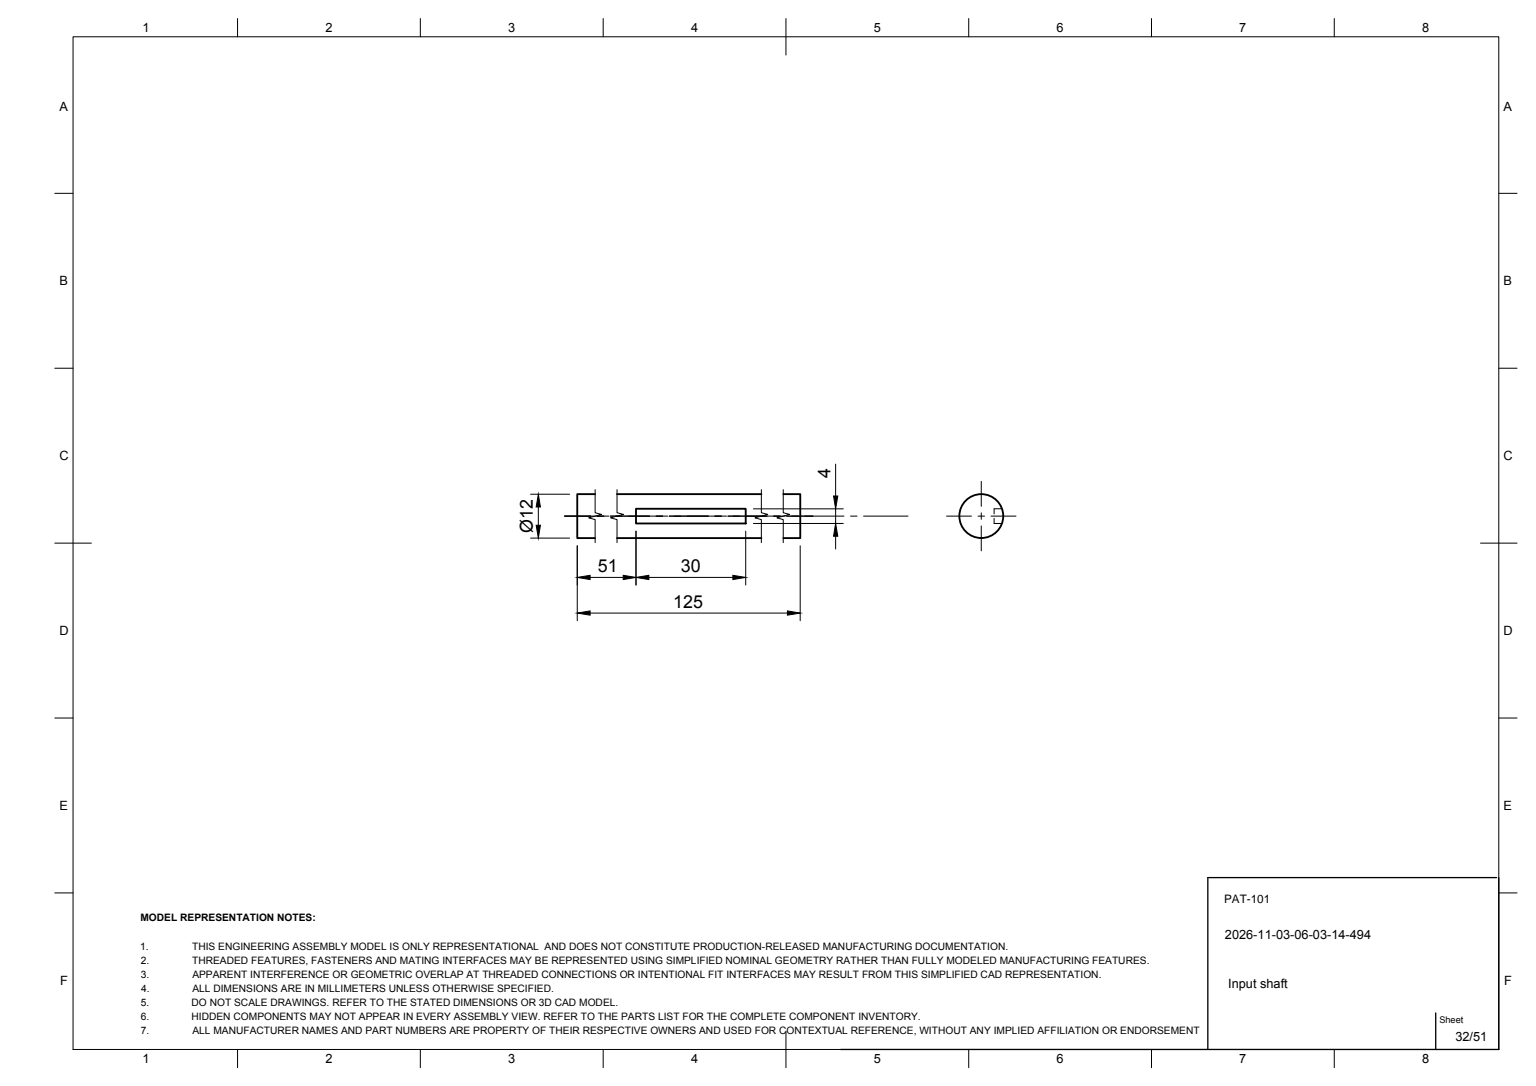
ISO-10303-21;
HEADER;
/* Generated by software containing ST-Developer
 * from STEP Tools, Inc. (www.steptools.com) 
 */

FILE_DESCRIPTION(
/* description */ ('Spur gear reduction stage 2-1 on bearing plates'),
/* implementation_level */ '2;1');

FILE_NAME(
/* name */ 'Input shaft.step',
/* time_stamp */ '2026-10-28T03:22:07-07:00',
/* author */ (''),
/* organization */ (''),
/* preprocessor_version */ 'ST-DEVELOPER v20.2',
/* originating_system */ 'Autodesk Translation Framework v15.17.0.0',
/* authorisation */ '');

FILE_SCHEMA (('AUTOMOTIVE_DESIGN { 1 0 10303 214 3 1 1 }'));
ENDSEC;

DATA;
#10=MECHANICAL_DESIGN_GEOMETRIC_PRESENTATION_REPRESENTATION('',(#986),#53909);
#885=SHAPE_REPRESENTATION_RELATIONSHIP('SRR','None',#54115,#928);
#928=ADVANCED_BREP_SHAPE_REPRESENTATION('',(#1041),#53889);
#986=STYLED_ITEM('',(#54397),#1041);
#1041=MANIFOLD_SOLID_BREP('Body1',#11313);
#1197=FACE_BOUND('',#2574,.T.);
#1358=PLANE('',#12482);
#1359=PLANE('',#12483);
#1360=PLANE('',#12485);
#1361=PLANE('',#12486);
#1362=PLANE('',#12487);
#1363=PLANE('',#12492);
#1364=PLANE('',#12493);
#1783=FACE_OUTER_BOUND('',#2568,.T.);
#1784=FACE_OUTER_BOUND('',#2569,.T.);
#1785=FACE_OUTER_BOUND('',#2570,.T.);
#1786=FACE_OUTER_BOUND('',#2571,.T.);
#1787=FACE_OUTER_BOUND('',#2572,.T.);
#1788=FACE_OUTER_BOUND('',#2573,.T.);
#1789=FACE_OUTER_BOUND('',#2575,.T.);
#1790=FACE_OUTER_BOUND('',#2576,.T.);
#2568=EDGE_LOOP('',(#8482,#8483,#8484,#8485));
#2569=EDGE_LOOP('',(#8486,#8487,#8488,#8489));
#2570=EDGE_LOOP('',(#8490,#8491,#8492,#8493));
#2571=EDGE_LOOP('',(#8494,#8495,#8496,#8497));
#2572=EDGE_LOOP('',(#8498,#8499,#8500,#8501));
#2573=EDGE_LOOP('',(#8502,#8503,#8504,#8505));
#2574=EDGE_LOOP('',(#8506,#8507,#8508,#8509));
#2575=EDGE_LOOP('',(#8510));
#2576=EDGE_LOOP('',(#8511));
#3193=LINE('',#17924,#3834);
#3194=LINE('',#17926,#3835);
#3195=LINE('',#17928,#3836);
#3196=LINE('',#17929,#3837);
#3197=LINE('',#17934,#3838);
#3198=LINE('',#17935,#3839);
#3199=LINE('',#17938,#3840);
#3200=LINE('',#17940,#3841);
#3201=LINE('',#17941,#3842);
#3202=LINE('',#17943,#3843);
#3203=LINE('',#17950,#3844);
#3834=VECTOR('',#14552,1.);
#3835=VECTOR('',#14553,1.);
#3836=VECTOR('',#14554,1.);
#3837=VECTOR('',#14555,1.);
#3838=VECTOR('',#14560,1.);
#3839=VECTOR('',#14561,1.);
#3840=VECTOR('',#14564,1.);
#3841=VECTOR('',#14565,1.);
#3842=VECTOR('',#14566,1.);
#3843=VECTOR('',#14569,1.);
#3844=VECTOR('',#14578,0.6);
#4576=CIRCLE('',#12484,0.6);
#4577=CIRCLE('',#12488,0.6);
#4578=CIRCLE('',#12490,0.6);
#4579=CIRCLE('',#12491,0.6);
#5174=VERTEX_POINT('',#17922);
#5175=VERTEX_POINT('',#17923);
#5176=VERTEX_POINT('',#17925);
#5177=VERTEX_POINT('',#17927);
#5178=VERTEX_POINT('',#17931);
#5179=VERTEX_POINT('',#17933);
#5180=VERTEX_POINT('',#17937);
#5181=VERTEX_POINT('',#17939);
#5182=VERTEX_POINT('',#17947);
#5183=VERTEX_POINT('',#17949);
#6383=EDGE_CURVE('',#5174,#5175,#3193,.T.);
#6384=EDGE_CURVE('',#5174,#5176,#3194,.T.);
#6385=EDGE_CURVE('',#5177,#5176,#3195,.T.);
#6386=EDGE_CURVE('',#5177,#5175,#3196,.T.);
#6387=EDGE_CURVE('',#5175,#5178,#4576,.T.);
#6388=EDGE_CURVE('',#5179,#5177,#3197,.T.);
#6389=EDGE_CURVE('',#5178,#5179,#3198,.T.);
#6390=EDGE_CURVE('',#5178,#5180,#3199,.T.);
#6391=EDGE_CURVE('',#5179,#5181,#3200,.T.);
#6392=EDGE_CURVE('',#5181,#5180,#3201,.T.);
#6393=EDGE_CURVE('',#5176,#5181,#3202,.T.);
#6394=EDGE_CURVE('',#5180,#5174,#4577,.T.);
#6395=EDGE_CURVE('',#5182,#5182,#4578,.T.);
#6396=EDGE_CURVE('',#5182,#5183,#3203,.T.);
#6397=EDGE_CURVE('',#5183,#5183,#4579,.T.);
#8482=ORIENTED_EDGE('',*,*,#6383,.F.);
#8483=ORIENTED_EDGE('',*,*,#6384,.T.);
#8484=ORIENTED_EDGE('',*,*,#6385,.F.);
#8485=ORIENTED_EDGE('',*,*,#6386,.T.);
#8486=ORIENTED_EDGE('',*,*,#6387,.F.);
#8487=ORIENTED_EDGE('',*,*,#6386,.F.);
#8488=ORIENTED_EDGE('',*,*,#6388,.F.);
#8489=ORIENTED_EDGE('',*,*,#6389,.F.);
#8490=ORIENTED_EDGE('',*,*,#6390,.F.);
#8491=ORIENTED_EDGE('',*,*,#6389,.T.);
#8492=ORIENTED_EDGE('',*,*,#6391,.T.);
#8493=ORIENTED_EDGE('',*,*,#6392,.T.);
#8494=ORIENTED_EDGE('',*,*,#6388,.T.);
#8495=ORIENTED_EDGE('',*,*,#6385,.T.);
#8496=ORIENTED_EDGE('',*,*,#6393,.T.);
#8497=ORIENTED_EDGE('',*,*,#6391,.F.);
#8498=ORIENTED_EDGE('',*,*,#6394,.F.);
#8499=ORIENTED_EDGE('',*,*,#6392,.F.);
#8500=ORIENTED_EDGE('',*,*,#6393,.F.);
#8501=ORIENTED_EDGE('',*,*,#6384,.F.);
#8502=ORIENTED_EDGE('',*,*,#6395,.F.);
#8503=ORIENTED_EDGE('',*,*,#6396,.T.);
#8504=ORIENTED_EDGE('',*,*,#6397,.T.);
#8505=ORIENTED_EDGE('',*,*,#6396,.F.);
#8506=ORIENTED_EDGE('',*,*,#6390,.T.);
#8507=ORIENTED_EDGE('',*,*,#6394,.T.);
#8508=ORIENTED_EDGE('',*,*,#6383,.T.);
#8509=ORIENTED_EDGE('',*,*,#6387,.T.);
#8510=ORIENTED_EDGE('',*,*,#6395,.T.);
#8511=ORIENTED_EDGE('',*,*,#6397,.F.);
#10526=CYLINDRICAL_SURFACE('',#12489,0.6);
#10903=ADVANCED_FACE('',(#1783),#1358,.F.);
#10904=ADVANCED_FACE('',(#1784),#1359,.T.);
#10905=ADVANCED_FACE('',(#1785),#1360,.F.);
#10906=ADVANCED_FACE('',(#1786),#1361,.F.);
#10907=ADVANCED_FACE('',(#1787),#1362,.F.);
#10908=ADVANCED_FACE('',(#1788,#1197),#10526,.T.);
#10909=ADVANCED_FACE('',(#1789),#1363,.T.);
#10910=ADVANCED_FACE('',(#1790),#1364,.F.);
#11313=CLOSED_SHELL('',(#10903,#10904,#10905,#10906,#10907,#10908,#10909,
#10910));
#12481=AXIS2_PLACEMENT_3D('',#17920,#14548,#14549);
#12482=AXIS2_PLACEMENT_3D('',#17921,#14550,#14551);
#12483=AXIS2_PLACEMENT_3D('',#17930,#14556,#14557);
#12484=AXIS2_PLACEMENT_3D('',#17932,#14558,#14559);
#12485=AXIS2_PLACEMENT_3D('',#17936,#14562,#14563);
#12486=AXIS2_PLACEMENT_3D('',#17942,#14567,#14568);
#12487=AXIS2_PLACEMENT_3D('',#17944,#14570,#14571);
#12488=AXIS2_PLACEMENT_3D('',#17945,#14572,#14573);
#12489=AXIS2_PLACEMENT_3D('',#17946,#14574,#14575);
#12490=AXIS2_PLACEMENT_3D('',#17948,#14576,#14577);
#12491=AXIS2_PLACEMENT_3D('',#17951,#14579,#14580);
#12492=AXIS2_PLACEMENT_3D('',#17952,#14581,#14582);
#12493=AXIS2_PLACEMENT_3D('',#17953,#14583,#14584);
#14548=DIRECTION('axis',(0.,0.,1.));
#14549=DIRECTION('refdir',(1.,0.,0.));
#14550=DIRECTION('center_axis',(-1.,0.,0.));
#14551=DIRECTION('ref_axis',(0.,0.,1.));
#14552=DIRECTION('',(0.,-1.,0.));
#14553=DIRECTION('',(0.,0.,1.));
#14554=DIRECTION('',(0.,1.,0.));
#14555=DIRECTION('',(0.,0.,-1.));
#14556=DIRECTION('center_axis',(0.,1.,0.));
#14557=DIRECTION('ref_axis',(1.,0.,0.));
#14558=DIRECTION('center_axis',(0.,-1.,0.));
#14559=DIRECTION('ref_axis',(1.,0.,0.));
#14560=DIRECTION('',(-1.,0.,0.));
#14561=DIRECTION('',(0.,0.,1.));
#14562=DIRECTION('center_axis',(1.,0.,0.));
#14563=DIRECTION('ref_axis',(0.,0.,-1.));
#14564=DIRECTION('',(0.,1.,0.));
#14565=DIRECTION('',(0.,1.,0.));
#14566=DIRECTION('',(0.,0.,-1.));
#14567=DIRECTION('center_axis',(0.,0.,1.));
#14568=DIRECTION('ref_axis',(1.,0.,0.));
#14569=DIRECTION('',(1.,0.,0.));
#14570=DIRECTION('center_axis',(0.,1.,0.));
#14571=DIRECTION('ref_axis',(0.,0.,1.));
#14572=DIRECTION('center_axis',(0.,1.,0.));
#14573=DIRECTION('ref_axis',(1.,0.,0.));
#14574=DIRECTION('center_axis',(0.,1.,0.));
#14575=DIRECTION('ref_axis',(1.,0.,0.));
#14576=DIRECTION('center_axis',(0.,1.,0.));
#14577=DIRECTION('ref_axis',(1.,0.,0.));
#14578=DIRECTION('',(0.,-1.,0.));
#14579=DIRECTION('center_axis',(0.,1.,0.));
#14580=DIRECTION('ref_axis',(1.,0.,0.));
#14581=DIRECTION('center_axis',(0.,1.,0.));
#14582=DIRECTION('ref_axis',(1.,0.,0.));
#14583=DIRECTION('center_axis',(0.,1.,0.));
#14584=DIRECTION('ref_axis',(1.,0.,0.));
#17920=CARTESIAN_POINT('',(0.,0.,0.));
#17921=CARTESIAN_POINT('Origin',(-0.2,-0.9,-0.7));
#17922=CARTESIAN_POINT('',(-0.2,2.1,-0.565685424949238));
#17923=CARTESIAN_POINT('',(-0.2,-0.9,-0.565685424949238));
#17924=CARTESIAN_POINT('',(-0.2,-6.,-0.565685424949238));
#17925=CARTESIAN_POINT('',(-0.2,2.1,-0.35));
#17926=CARTESIAN_POINT('',(-0.2,2.1,-0.35));
#17927=CARTESIAN_POINT('',(-0.2,-0.9,-0.35));
#17928=CARTESIAN_POINT('',(-0.2,-0.9,-0.35));
#17929=CARTESIAN_POINT('',(-0.2,-0.9,-0.35));
#17930=CARTESIAN_POINT('Origin',(0.,-0.9,-0.525));
#17931=CARTESIAN_POINT('',(0.2,-0.9,-0.565685424949238));
#17932=CARTESIAN_POINT('Origin',(0.,-0.9,0.));
#17933=CARTESIAN_POINT('',(0.2,-0.9,-0.35));
#17934=CARTESIAN_POINT('',(0.2,-0.9,-0.35));
#17935=CARTESIAN_POINT('',(0.2,-0.9,-0.7));
#17936=CARTESIAN_POINT('Origin',(0.2,-0.9,-0.35));
#17937=CARTESIAN_POINT('',(0.2,2.1,-0.565685424949238));
#17938=CARTESIAN_POINT('',(0.2,-6.,-0.565685424949238));
#17939=CARTESIAN_POINT('',(0.2,2.1,-0.35));
#17940=CARTESIAN_POINT('',(0.2,-0.9,-0.35));
#17941=CARTESIAN_POINT('',(0.2,2.1,-0.7));
#17942=CARTESIAN_POINT('Origin',(-0.2,-0.9,-0.35));
#17943=CARTESIAN_POINT('',(0.2,2.1,-0.35));
#17944=CARTESIAN_POINT('Origin',(0.,2.1,-0.525));
#17945=CARTESIAN_POINT('Origin',(0.,2.1,0.));
#17946=CARTESIAN_POINT('Origin',(0.,-6.,0.));
#17947=CARTESIAN_POINT('',(-0.6,6.5,7.34788079488412E-17));
#17948=CARTESIAN_POINT('Origin',(0.,6.5,0.));
#17949=CARTESIAN_POINT('',(-0.6,-6.,7.34788079488412E-17));
#17950=CARTESIAN_POINT('',(-0.6,-6.,7.34788079488412E-17));
#17951=CARTESIAN_POINT('Origin',(0.,-6.,0.));
#17952=CARTESIAN_POINT('Origin',(0.,6.5,0.));
#17953=CARTESIAN_POINT('Origin',(0.,-6.,0.));
#53839=UNCERTAINTY_MEASURE_WITH_UNIT(LENGTH_MEASURE(0.001),#53910,
'DISTANCE_ACCURACY_VALUE',
'Maximum model space distance between geometric entities at asserted c
onnectivities');
#53859=UNCERTAINTY_MEASURE_WITH_UNIT(LENGTH_MEASURE(0.001),#53910,
'DISTANCE_ACCURACY_VALUE',
'Maximum model space distance between geometric entities at asserted c
onnectivities');
#53889=(
GEOMETRIC_REPRESENTATION_CONTEXT(3)
GLOBAL_UNCERTAINTY_ASSIGNED_CONTEXT((#53839))
GLOBAL_UNIT_ASSIGNED_CONTEXT((#53910,#53912,#53913))
REPRESENTATION_CONTEXT('','3D')
);
#53909=(
GEOMETRIC_REPRESENTATION_CONTEXT(3)
GLOBAL_UNCERTAINTY_ASSIGNED_CONTEXT((#53859))
GLOBAL_UNIT_ASSIGNED_CONTEXT((#53910,#53912,#53913))
REPRESENTATION_CONTEXT('','3D')
);
#53910=(
LENGTH_UNIT()
NAMED_UNIT(*)
SI_UNIT(.CENTI.,.METRE.)
);
#53912=(
NAMED_UNIT(*)
PLANE_ANGLE_UNIT()
SI_UNIT($,.RADIAN.)
);
#53913=(
NAMED_UNIT(*)
SI_UNIT($,.STERADIAN.)
SOLID_ANGLE_UNIT()
);
#53943=SHAPE_DEFINITION_REPRESENTATION(#54041,#54115);
#54041=PRODUCT_DEFINITION_SHAPE('',$,#54165);
#54115=SHAPE_REPRESENTATION('',(#12481),#53889);
#54135=PRODUCT_DEFINITION_CONTEXT('part definition',#54284,'design');
#54165=PRODUCT_DEFINITION('Input shaft','Input shaft',#54214,#54135);
#54214=PRODUCT_DEFINITION_FORMATION('',$,#54315);
#54284=APPLICATION_CONTEXT(
'Core Data for Automotive Mechanical Design Process');
#54285=PRODUCT_CONTEXT('part definition',#54284,'mechanical');
#54315=PRODUCT('Input shaft','Input shaft','Input shaft',(#54285));
#54391=COLOUR_RGB('Grey',0.48,0.52,0.57);
#54392=FILL_AREA_STYLE_COLOUR('',#54391);
#54393=FILL_AREA_STYLE('',(#54392));
#54394=SURFACE_STYLE_FILL_AREA(#54393);
#54395=SURFACE_SIDE_STYLE('',(#54394));
#54396=SURFACE_STYLE_USAGE(.BOTH.,#54395);
#54397=PRESENTATION_STYLE_ASSIGNMENT((#54396));
ENDSEC;
END-ISO-10303-21;
